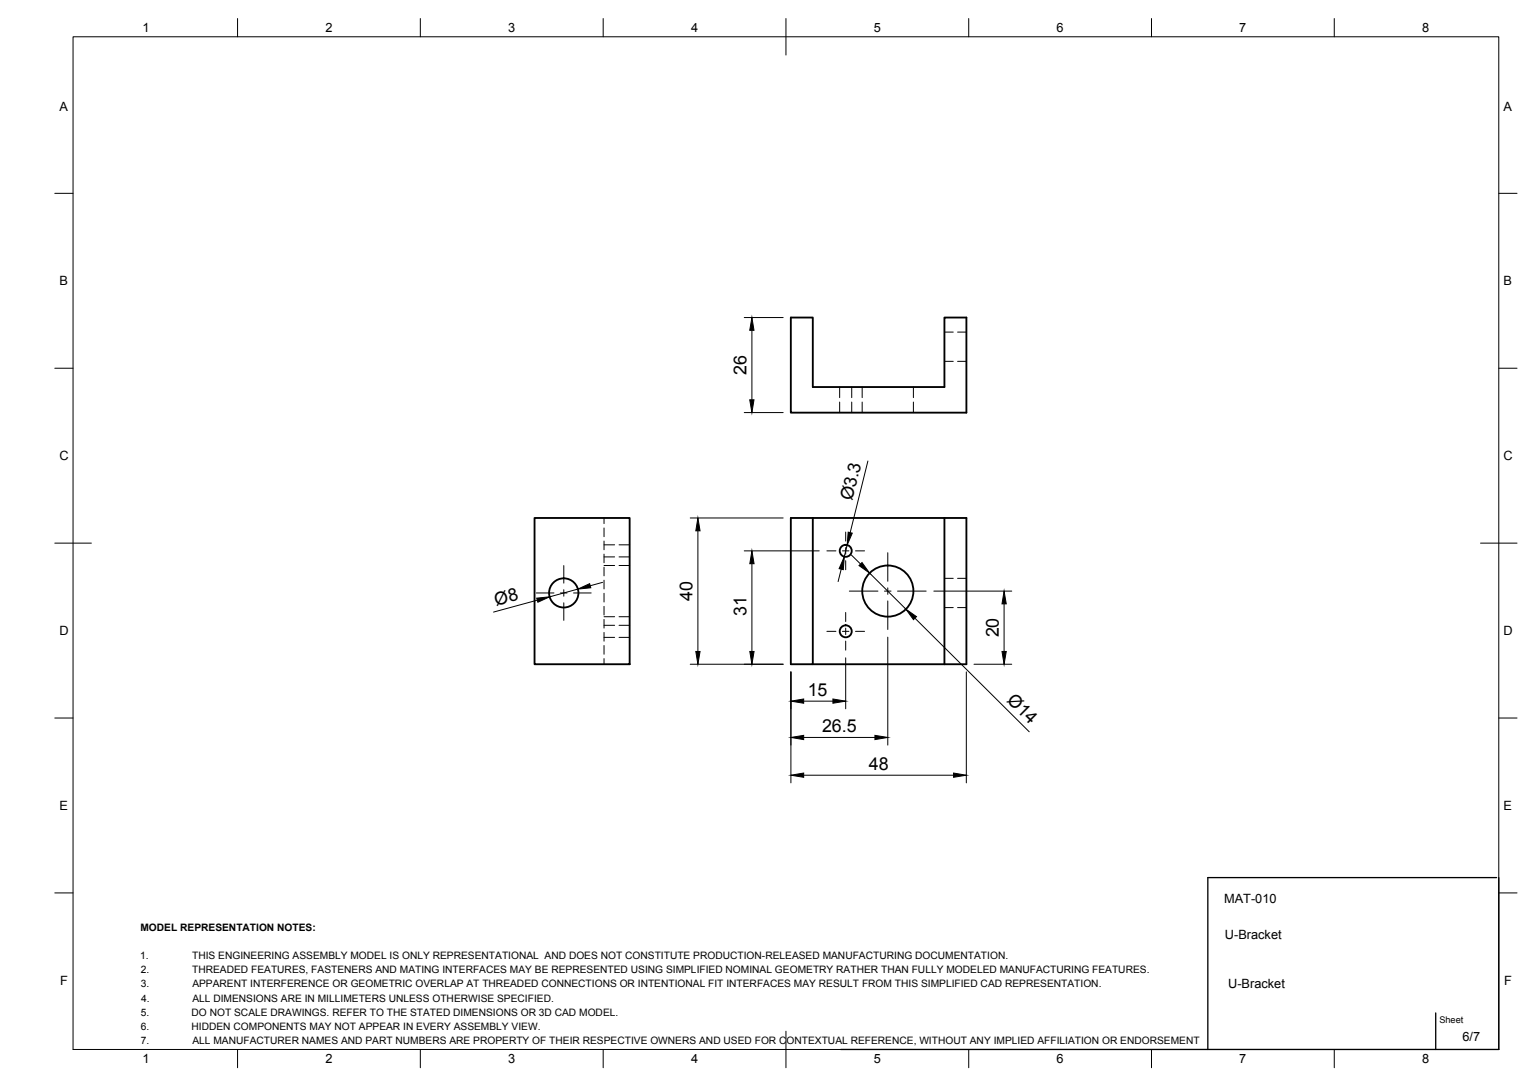
ISO-10303-21;
HEADER;
/* Generated by software containing ST-Developer
 * from STEP Tools, Inc. (www.steptools.com) 
 */

FILE_DESCRIPTION(
/* description */ ('STEP AP214'),
/* implementation_level */ '2;1');

FILE_NAME(
/* name */ 'U-Bracket.step',
/* time_stamp */ '2026-11-14T05:50:49-08:00',
/* author */ (''),
/* organization */ (''),
/* preprocessor_version */ 'ST-DEVELOPER v20.2',
/* originating_system */ 'Autodesk Translation Framework v15.17.0.0',
/* authorisation */ '');

FILE_SCHEMA (('AUTOMOTIVE_DESIGN { 1 0 10303 214 3 1 1 }'));
ENDSEC;

DATA;
#10=MECHANICAL_DESIGN_GEOMETRIC_PRESENTATION_REPRESENTATION('',(#161),#9903);
#147=SHAPE_REPRESENTATION_RELATIONSHIP('SRR','None',#9942,#154);
#154=ADVANCED_BREP_SHAPE_REPRESENTATION('',(#168),#9900);
#161=STYLED_ITEM('',(#9982),#168);
#168=MANIFOLD_SOLID_BREP('Body1',#2026);
#183=FACE_BOUND('',#426,.T.);
#184=FACE_BOUND('',#427,.T.);
#185=FACE_BOUND('',#428,.T.);
#186=FACE_BOUND('',#430,.T.);
#187=FACE_BOUND('',#435,.T.);
#188=FACE_BOUND('',#436,.T.);
#189=FACE_BOUND('',#437,.T.);
#190=FACE_BOUND('',#441,.T.);
#214=PLANE('',#2211);
#215=PLANE('',#2212);
#216=PLANE('',#2213);
#217=PLANE('',#2214);
#218=PLANE('',#2215);
#219=PLANE('',#2216);
#220=PLANE('',#2217);
#221=PLANE('',#2218);
#222=PLANE('',#2219);
#223=PLANE('',#2220);
#291=FACE_OUTER_BOUND('',#421,.T.);
#292=FACE_OUTER_BOUND('',#422,.T.);
#293=FACE_OUTER_BOUND('',#423,.T.);
#294=FACE_OUTER_BOUND('',#424,.T.);
#295=FACE_OUTER_BOUND('',#425,.T.);
#296=FACE_OUTER_BOUND('',#429,.T.);
#297=FACE_OUTER_BOUND('',#431,.T.);
#298=FACE_OUTER_BOUND('',#432,.T.);
#299=FACE_OUTER_BOUND('',#433,.T.);
#300=FACE_OUTER_BOUND('',#434,.T.);
#301=FACE_OUTER_BOUND('',#438,.T.);
#302=FACE_OUTER_BOUND('',#439,.T.);
#303=FACE_OUTER_BOUND('',#440,.T.);
#304=FACE_OUTER_BOUND('',#442,.T.);
#421=EDGE_LOOP('',(#1448,#1449,#1450,#1451));
#422=EDGE_LOOP('',(#1452,#1453,#1454,#1455));
#423=EDGE_LOOP('',(#1456,#1457,#1458,#1459));
#424=EDGE_LOOP('',(#1460,#1461,#1462,#1463));
#425=EDGE_LOOP('',(#1464,#1465,#1466,#1467));
#426=EDGE_LOOP('',(#1468));
#427=EDGE_LOOP('',(#1469));
#428=EDGE_LOOP('',(#1470));
#429=EDGE_LOOP('',(#1471,#1472,#1473,#1474));
#430=EDGE_LOOP('',(#1475));
#431=EDGE_LOOP('',(#1476,#1477,#1478,#1479,#1480,#1481,#1482,#1483));
#432=EDGE_LOOP('',(#1484,#1485,#1486,#1487));
#433=EDGE_LOOP('',(#1488,#1489,#1490,#1491,#1492,#1493,#1494,#1495));
#434=EDGE_LOOP('',(#1496,#1497,#1498,#1499));
#435=EDGE_LOOP('',(#1500));
#436=EDGE_LOOP('',(#1501));
#437=EDGE_LOOP('',(#1502));
#438=EDGE_LOOP('',(#1503,#1504,#1505,#1506));
#439=EDGE_LOOP('',(#1507,#1508,#1509,#1510));
#440=EDGE_LOOP('',(#1511,#1512,#1513,#1514));
#441=EDGE_LOOP('',(#1515));
#442=EDGE_LOOP('',(#1516,#1517,#1518,#1519));
#535=LINE('',#3038,#671);
#536=LINE('',#3044,#672);
#537=LINE('',#3050,#673);
#538=LINE('',#3056,#674);
#539=LINE('',#3061,#675);
#540=LINE('',#3063,#676);
#541=LINE('',#3065,#677);
#542=LINE('',#3066,#678);
#543=LINE('',#3070,#679);
#544=LINE('',#3072,#680);
#545=LINE('',#3074,#681);
#546=LINE('',#3075,#682);
#547=LINE('',#3078,#683);
#548=LINE('',#3080,#684);
#549=LINE('',#3082,#685);
#550=LINE('',#3083,#686);
#551=LINE('',#3085,#687);
#552=LINE('',#3086,#688);
#553=LINE('',#3089,#689);
#554=LINE('',#3091,#690);
#555=LINE('',#3092,#691);
#556=LINE('',#3094,#692);
#557=LINE('',#3096,#693);
#558=LINE('',#3097,#694);
#559=LINE('',#3099,#695);
#560=LINE('',#3100,#696);
#561=LINE('',#3103,#697);
#562=LINE('',#3106,#698);
#671=VECTOR('',#2528,4.);
#672=VECTOR('',#2535,1.64999999999999);
#673=VECTOR('',#2542,1.64999999999999);
#674=VECTOR('',#2549,7.);
#675=VECTOR('',#2554,1000.);
#676=VECTOR('',#2555,1000.);
#677=VECTOR('',#2556,1000.);
#678=VECTOR('',#2557,1000.);
#679=VECTOR('',#2560,1000.);
#680=VECTOR('',#2561,1000.);
#681=VECTOR('',#2562,1000.);
#682=VECTOR('',#2563,1000.);
#683=VECTOR('',#2566,1000.);
#684=VECTOR('',#2567,1000.);
#685=VECTOR('',#2568,1000.);
#686=VECTOR('',#2569,1000.);
#687=VECTOR('',#2570,1000.);
#688=VECTOR('',#2571,1000.);
#689=VECTOR('',#2574,1000.);
#690=VECTOR('',#2575,1000.);
#691=VECTOR('',#2576,1000.);
#692=VECTOR('',#2579,1000.);
#693=VECTOR('',#2580,1000.);
#694=VECTOR('',#2581,1000.);
#695=VECTOR('',#2582,1000.);
#696=VECTOR('',#2583,1000.);
#697=VECTOR('',#2588,1000.);
#698=VECTOR('',#2593,1000.);
#832=CIRCLE('',#2200,4.);
#833=CIRCLE('',#2201,4.);
#834=CIRCLE('',#2203,1.64999999999999);
#835=CIRCLE('',#2204,1.64999999999999);
#836=CIRCLE('',#2206,1.64999999999999);
#837=CIRCLE('',#2207,1.64999999999999);
#838=CIRCLE('',#2209,7.);
#839=CIRCLE('',#2210,7.);
#903=VERTEX_POINT('',#3035);
#904=VERTEX_POINT('',#3037);
#905=VERTEX_POINT('',#3041);
#906=VERTEX_POINT('',#3043);
#907=VERTEX_POINT('',#3047);
#908=VERTEX_POINT('',#3049);
#909=VERTEX_POINT('',#3053);
#910=VERTEX_POINT('',#3055);
#911=VERTEX_POINT('',#3059);
#912=VERTEX_POINT('',#3060);
#913=VERTEX_POINT('',#3062);
#914=VERTEX_POINT('',#3064);
#915=VERTEX_POINT('',#3068);
#916=VERTEX_POINT('',#3069);
#917=VERTEX_POINT('',#3071);
#918=VERTEX_POINT('',#3073);
#919=VERTEX_POINT('',#3077);
#920=VERTEX_POINT('',#3079);
#921=VERTEX_POINT('',#3081);
#922=VERTEX_POINT('',#3084);
#923=VERTEX_POINT('',#3088);
#924=VERTEX_POINT('',#3090);
#925=VERTEX_POINT('',#3095);
#926=VERTEX_POINT('',#3098);
#1105=EDGE_CURVE('',#903,#903,#832,.T.);
#1106=EDGE_CURVE('',#903,#904,#535,.T.);
#1107=EDGE_CURVE('',#904,#904,#833,.T.);
#1108=EDGE_CURVE('',#905,#905,#834,.T.);
#1109=EDGE_CURVE('',#905,#906,#536,.T.);
#1110=EDGE_CURVE('',#906,#906,#835,.T.);
#1111=EDGE_CURVE('',#907,#907,#836,.T.);
#1112=EDGE_CURVE('',#907,#908,#537,.T.);
#1113=EDGE_CURVE('',#908,#908,#837,.T.);
#1114=EDGE_CURVE('',#909,#909,#838,.T.);
#1115=EDGE_CURVE('',#909,#910,#538,.T.);
#1116=EDGE_CURVE('',#910,#910,#839,.T.);
#1117=EDGE_CURVE('',#911,#912,#539,.T.);
#1118=EDGE_CURVE('',#913,#912,#540,.T.);
#1119=EDGE_CURVE('',#913,#914,#541,.T.);
#1120=EDGE_CURVE('',#911,#914,#542,.T.);
#1121=EDGE_CURVE('',#915,#916,#543,.T.);
#1122=EDGE_CURVE('',#917,#916,#544,.T.);
#1123=EDGE_CURVE('',#918,#917,#545,.T.);
#1124=EDGE_CURVE('',#918,#915,#546,.T.);
#1125=EDGE_CURVE('',#916,#919,#547,.T.);
#1126=EDGE_CURVE('',#920,#919,#548,.T.);
#1127=EDGE_CURVE('',#921,#920,#549,.T.);
#1128=EDGE_CURVE('',#921,#914,#550,.T.);
#1129=EDGE_CURVE('',#922,#913,#551,.T.);
#1130=EDGE_CURVE('',#917,#922,#552,.T.);
#1131=EDGE_CURVE('',#919,#923,#553,.T.);
#1132=EDGE_CURVE('',#924,#923,#554,.T.);
#1133=EDGE_CURVE('',#920,#924,#555,.T.);
#1134=EDGE_CURVE('',#923,#915,#556,.T.);
#1135=EDGE_CURVE('',#925,#918,#557,.T.);
#1136=EDGE_CURVE('',#925,#912,#558,.T.);
#1137=EDGE_CURVE('',#926,#911,#559,.T.);
#1138=EDGE_CURVE('',#924,#926,#560,.T.);
#1139=EDGE_CURVE('',#926,#921,#561,.T.);
#1140=EDGE_CURVE('',#922,#925,#562,.T.);
#1448=ORIENTED_EDGE('',*,*,#1105,.F.);
#1449=ORIENTED_EDGE('',*,*,#1106,.T.);
#1450=ORIENTED_EDGE('',*,*,#1107,.T.);
#1451=ORIENTED_EDGE('',*,*,#1106,.F.);
#1452=ORIENTED_EDGE('',*,*,#1108,.T.);
#1453=ORIENTED_EDGE('',*,*,#1109,.T.);
#1454=ORIENTED_EDGE('',*,*,#1110,.T.);
#1455=ORIENTED_EDGE('',*,*,#1109,.F.);
#1456=ORIENTED_EDGE('',*,*,#1111,.T.);
#1457=ORIENTED_EDGE('',*,*,#1112,.T.);
#1458=ORIENTED_EDGE('',*,*,#1113,.T.);
#1459=ORIENTED_EDGE('',*,*,#1112,.F.);
#1460=ORIENTED_EDGE('',*,*,#1114,.T.);
#1461=ORIENTED_EDGE('',*,*,#1115,.T.);
#1462=ORIENTED_EDGE('',*,*,#1116,.T.);
#1463=ORIENTED_EDGE('',*,*,#1115,.F.);
#1464=ORIENTED_EDGE('',*,*,#1117,.T.);
#1465=ORIENTED_EDGE('',*,*,#1118,.F.);
#1466=ORIENTED_EDGE('',*,*,#1119,.T.);
#1467=ORIENTED_EDGE('',*,*,#1120,.F.);
#1468=ORIENTED_EDGE('',*,*,#1108,.F.);
#1469=ORIENTED_EDGE('',*,*,#1111,.F.);
#1470=ORIENTED_EDGE('',*,*,#1114,.F.);
#1471=ORIENTED_EDGE('',*,*,#1121,.T.);
#1472=ORIENTED_EDGE('',*,*,#1122,.F.);
#1473=ORIENTED_EDGE('',*,*,#1123,.F.);
#1474=ORIENTED_EDGE('',*,*,#1124,.T.);
#1475=ORIENTED_EDGE('',*,*,#1107,.F.);
#1476=ORIENTED_EDGE('',*,*,#1125,.T.);
#1477=ORIENTED_EDGE('',*,*,#1126,.F.);
#1478=ORIENTED_EDGE('',*,*,#1127,.F.);
#1479=ORIENTED_EDGE('',*,*,#1128,.T.);
#1480=ORIENTED_EDGE('',*,*,#1119,.F.);
#1481=ORIENTED_EDGE('',*,*,#1129,.F.);
#1482=ORIENTED_EDGE('',*,*,#1130,.F.);
#1483=ORIENTED_EDGE('',*,*,#1122,.T.);
#1484=ORIENTED_EDGE('',*,*,#1131,.T.);
#1485=ORIENTED_EDGE('',*,*,#1132,.F.);
#1486=ORIENTED_EDGE('',*,*,#1133,.F.);
#1487=ORIENTED_EDGE('',*,*,#1126,.T.);
#1488=ORIENTED_EDGE('',*,*,#1134,.T.);
#1489=ORIENTED_EDGE('',*,*,#1124,.F.);
#1490=ORIENTED_EDGE('',*,*,#1135,.F.);
#1491=ORIENTED_EDGE('',*,*,#1136,.T.);
#1492=ORIENTED_EDGE('',*,*,#1117,.F.);
#1493=ORIENTED_EDGE('',*,*,#1137,.F.);
#1494=ORIENTED_EDGE('',*,*,#1138,.F.);
#1495=ORIENTED_EDGE('',*,*,#1132,.T.);
#1496=ORIENTED_EDGE('',*,*,#1121,.F.);
#1497=ORIENTED_EDGE('',*,*,#1134,.F.);
#1498=ORIENTED_EDGE('',*,*,#1131,.F.);
#1499=ORIENTED_EDGE('',*,*,#1125,.F.);
#1500=ORIENTED_EDGE('',*,*,#1110,.F.);
#1501=ORIENTED_EDGE('',*,*,#1113,.F.);
#1502=ORIENTED_EDGE('',*,*,#1116,.F.);
#1503=ORIENTED_EDGE('',*,*,#1120,.T.);
#1504=ORIENTED_EDGE('',*,*,#1128,.F.);
#1505=ORIENTED_EDGE('',*,*,#1139,.F.);
#1506=ORIENTED_EDGE('',*,*,#1137,.T.);
#1507=ORIENTED_EDGE('',*,*,#1133,.T.);
#1508=ORIENTED_EDGE('',*,*,#1138,.T.);
#1509=ORIENTED_EDGE('',*,*,#1139,.T.);
#1510=ORIENTED_EDGE('',*,*,#1127,.T.);
#1511=ORIENTED_EDGE('',*,*,#1118,.T.);
#1512=ORIENTED_EDGE('',*,*,#1136,.F.);
#1513=ORIENTED_EDGE('',*,*,#1140,.F.);
#1514=ORIENTED_EDGE('',*,*,#1129,.T.);
#1515=ORIENTED_EDGE('',*,*,#1105,.T.);
#1516=ORIENTED_EDGE('',*,*,#1123,.T.);
#1517=ORIENTED_EDGE('',*,*,#1130,.T.);
#1518=ORIENTED_EDGE('',*,*,#1140,.T.);
#1519=ORIENTED_EDGE('',*,*,#1135,.T.);
#1870=CYLINDRICAL_SURFACE('',#2199,4.);
#1871=CYLINDRICAL_SURFACE('',#2202,1.64999999999999);
#1872=CYLINDRICAL_SURFACE('',#2205,1.64999999999999);
#1873=CYLINDRICAL_SURFACE('',#2208,7.);
#1943=ADVANCED_FACE('',(#291),#1870,.F.);
#1944=ADVANCED_FACE('',(#292),#1871,.F.);
#1945=ADVANCED_FACE('',(#293),#1872,.F.);
#1946=ADVANCED_FACE('',(#294),#1873,.F.);
#1947=ADVANCED_FACE('',(#295,#183,#184,#185),#214,.T.);
#1948=ADVANCED_FACE('',(#296,#186),#215,.F.);
#1949=ADVANCED_FACE('',(#297),#216,.F.);
#1950=ADVANCED_FACE('',(#298),#217,.F.);
#1951=ADVANCED_FACE('',(#299),#218,.F.);
#1952=ADVANCED_FACE('',(#300,#187,#188,#189),#219,.F.);
#1953=ADVANCED_FACE('',(#301),#220,.F.);
#1954=ADVANCED_FACE('',(#302),#221,.T.);
#1955=ADVANCED_FACE('',(#303,#190),#222,.F.);
#1956=ADVANCED_FACE('',(#304),#223,.F.);
#2026=CLOSED_SHELL('',(#1943,#1944,#1945,#1946,#1947,#1948,#1949,#1950,
#1951,#1952,#1953,#1954,#1955,#1956));
#2198=AXIS2_PLACEMENT_3D('',#3033,#2522,#2523);
#2199=AXIS2_PLACEMENT_3D('',#3034,#2524,#2525);
#2200=AXIS2_PLACEMENT_3D('',#3036,#2526,#2527);
#2201=AXIS2_PLACEMENT_3D('',#3039,#2529,#2530);
#2202=AXIS2_PLACEMENT_3D('',#3040,#2531,#2532);
#2203=AXIS2_PLACEMENT_3D('',#3042,#2533,#2534);
#2204=AXIS2_PLACEMENT_3D('',#3045,#2536,#2537);
#2205=AXIS2_PLACEMENT_3D('',#3046,#2538,#2539);
#2206=AXIS2_PLACEMENT_3D('',#3048,#2540,#2541);
#2207=AXIS2_PLACEMENT_3D('',#3051,#2543,#2544);
#2208=AXIS2_PLACEMENT_3D('',#3052,#2545,#2546);
#2209=AXIS2_PLACEMENT_3D('',#3054,#2547,#2548);
#2210=AXIS2_PLACEMENT_3D('',#3057,#2550,#2551);
#2211=AXIS2_PLACEMENT_3D('',#3058,#2552,#2553);
#2212=AXIS2_PLACEMENT_3D('',#3067,#2558,#2559);
#2213=AXIS2_PLACEMENT_3D('',#3076,#2564,#2565);
#2214=AXIS2_PLACEMENT_3D('',#3087,#2572,#2573);
#2215=AXIS2_PLACEMENT_3D('',#3093,#2577,#2578);
#2216=AXIS2_PLACEMENT_3D('',#3101,#2584,#2585);
#2217=AXIS2_PLACEMENT_3D('',#3102,#2586,#2587);
#2218=AXIS2_PLACEMENT_3D('',#3104,#2589,#2590);
#2219=AXIS2_PLACEMENT_3D('',#3105,#2591,#2592);
#2220=AXIS2_PLACEMENT_3D('',#3107,#2594,#2595);
#2522=DIRECTION('axis',(0.,0.,1.));
#2523=DIRECTION('refdir',(1.,0.,0.));
#2524=DIRECTION('center_axis',(0.,-1.,0.));
#2525=DIRECTION('ref_axis',(0.,0.,-1.));
#2526=DIRECTION('center_axis',(0.,-1.,0.));
#2527=DIRECTION('ref_axis',(0.,0.,-1.));
#2528=DIRECTION('',(0.,-1.,0.));
#2529=DIRECTION('center_axis',(0.,-1.,0.));
#2530=DIRECTION('ref_axis',(0.,0.,-1.));
#2531=DIRECTION('center_axis',(0.,0.,-1.));
#2532=DIRECTION('ref_axis',(-1.,0.,0.));
#2533=DIRECTION('center_axis',(0.,0.,1.));
#2534=DIRECTION('ref_axis',(1.,0.,0.));
#2535=DIRECTION('',(0.,0.,-1.));
#2536=DIRECTION('center_axis',(0.,0.,-1.));
#2537=DIRECTION('ref_axis',(-1.,0.,0.));
#2538=DIRECTION('center_axis',(0.,0.,-1.));
#2539=DIRECTION('ref_axis',(-1.,0.,0.));
#2540=DIRECTION('center_axis',(0.,0.,1.));
#2541=DIRECTION('ref_axis',(1.,0.,0.));
#2542=DIRECTION('',(0.,0.,-1.));
#2543=DIRECTION('center_axis',(0.,0.,-1.));
#2544=DIRECTION('ref_axis',(-1.,0.,0.));
#2545=DIRECTION('center_axis',(0.,0.,-1.));
#2546=DIRECTION('ref_axis',(-1.,0.,0.));
#2547=DIRECTION('center_axis',(0.,0.,1.));
#2548=DIRECTION('ref_axis',(1.,0.,0.));
#2549=DIRECTION('',(0.,0.,-1.));
#2550=DIRECTION('center_axis',(0.,0.,-1.));
#2551=DIRECTION('ref_axis',(-1.,0.,0.));
#2552=DIRECTION('center_axis',(0.,0.,1.));
#2553=DIRECTION('ref_axis',(1.,0.,0.));
#2554=DIRECTION('',(0.,-1.,0.));
#2555=DIRECTION('',(-1.,0.,0.));
#2556=DIRECTION('',(0.,1.,0.));
#2557=DIRECTION('',(1.,0.,0.));
#2558=DIRECTION('center_axis',(0.,1.,0.));
#2559=DIRECTION('ref_axis',(0.,0.,1.));
#2560=DIRECTION('',(1.,0.,0.));
#2561=DIRECTION('',(0.,0.,-1.));
#2562=DIRECTION('',(1.,0.,0.));
#2563=DIRECTION('',(0.,0.,-1.));
#2564=DIRECTION('center_axis',(-1.,0.,0.));
#2565=DIRECTION('ref_axis',(0.,0.,1.));
#2566=DIRECTION('',(0.,1.,0.));
#2567=DIRECTION('',(0.,0.,-1.));
#2568=DIRECTION('',(0.,1.,0.));
#2569=DIRECTION('',(0.,0.,-1.));
#2570=DIRECTION('',(0.,0.,-1.));
#2571=DIRECTION('',(0.,1.,0.));
#2572=DIRECTION('center_axis',(8.67361737988404E-17,-1.,0.));
#2573=DIRECTION('ref_axis',(1.,8.67361737988404E-17,0.));
#2574=DIRECTION('',(-1.,-8.67361737988404E-17,0.));
#2575=DIRECTION('',(0.,0.,-1.));
#2576=DIRECTION('',(-1.,-8.67361737988404E-17,0.));
#2577=DIRECTION('center_axis',(1.,0.,0.));
#2578=DIRECTION('ref_axis',(0.,0.,-1.));
#2579=DIRECTION('',(0.,-1.,0.));
#2580=DIRECTION('',(0.,-1.,0.));
#2581=DIRECTION('',(0.,0.,-1.));
#2582=DIRECTION('',(0.,0.,-1.));
#2583=DIRECTION('',(0.,-1.,0.));
#2584=DIRECTION('center_axis',(0.,0.,1.));
#2585=DIRECTION('ref_axis',(1.,0.,0.));
#2586=DIRECTION('center_axis',(0.,1.,0.));
#2587=DIRECTION('ref_axis',(0.,0.,1.));
#2588=DIRECTION('',(1.,0.,0.));
#2589=DIRECTION('center_axis',(0.,0.,1.));
#2590=DIRECTION('ref_axis',(1.,0.,0.));
#2591=DIRECTION('center_axis',(0.,-1.,0.));
#2592=DIRECTION('ref_axis',(0.,0.,-1.));
#2593=DIRECTION('',(-1.,0.,0.));
#2594=DIRECTION('center_axis',(0.,0.,-1.));
#2595=DIRECTION('ref_axis',(-1.,0.,0.));
#3033=CARTESIAN_POINT('',(0.,0.,0.));
#3034=CARTESIAN_POINT('Origin',(-0.506247771123191,-14.,18.0160339934195));
#3035=CARTESIAN_POINT('',(-0.506247771123192,-18.,22.0160339934195));
#3036=CARTESIAN_POINT('Origin',(-0.506247771123191,-18.,18.0160339934195));
#3037=CARTESIAN_POINT('',(-0.506247771123192,-24.,22.0160339934195));
#3038=CARTESIAN_POINT('',(-0.506247771123192,-14.,22.0160339934195));
#3039=CARTESIAN_POINT('Origin',(-0.506247771123191,-24.,18.0160339934195));
#3040=CARTESIAN_POINT('Origin',(-11.,9.00000000000001,0.));
#3041=CARTESIAN_POINT('',(-9.35000000000001,9.00000000000001,7.));
#3042=CARTESIAN_POINT('Origin',(-11.,9.00000000000001,7.));
#3043=CARTESIAN_POINT('',(-9.35000000000001,9.00000000000001,-1.35323471305782E-15));
#3044=CARTESIAN_POINT('',(-9.35000000000001,9.00000000000001,0.));
#3045=CARTESIAN_POINT('Origin',(-11.,9.00000000000001,-1.35323471305782E-15));
#3046=CARTESIAN_POINT('Origin',(11.,9.,0.));
#3047=CARTESIAN_POINT('',(12.65,9.,7.));
#3048=CARTESIAN_POINT('Origin',(11.,9.,7.));
#3049=CARTESIAN_POINT('',(12.65,9.,-1.35323471305782E-15));
#3050=CARTESIAN_POINT('',(12.65,9.,0.));
#3051=CARTESIAN_POINT('Origin',(11.,9.,-1.35323471305782E-15));
#3052=CARTESIAN_POINT('Origin',(0.,-2.5,9.99999999999999));
#3053=CARTESIAN_POINT('',(7.,-2.5,7.));
#3054=CARTESIAN_POINT('Origin',(0.,-2.5,7.));
#3055=CARTESIAN_POINT('',(7.,-2.5,-1.11022302462516E-15));
#3056=CARTESIAN_POINT('',(7.,-2.5,9.99999999999999));
#3057=CARTESIAN_POINT('Origin',(0.,-2.5,0.));
#3058=CARTESIAN_POINT('Origin',(0.,0.,7.));
#3059=CARTESIAN_POINT('',(-20.,18.,7.));
#3060=CARTESIAN_POINT('',(-20.,-18.,7.));
#3061=CARTESIAN_POINT('',(-20.,24.,7.));
#3062=CARTESIAN_POINT('',(20.,-18.,7.));
#3063=CARTESIAN_POINT('',(-20.,-18.,7.));
#3064=CARTESIAN_POINT('',(20.,18.,7.));
#3065=CARTESIAN_POINT('',(20.,-24.,7.));
#3066=CARTESIAN_POINT('',(-20.,18.,7.));
#3067=CARTESIAN_POINT('Origin',(2.93915231795365E-15,-24.,7.));
#3068=CARTESIAN_POINT('',(-20.,-24.,0.));
#3069=CARTESIAN_POINT('',(20.,-24.,0.));
#3070=CARTESIAN_POINT('',(2.93915231795365E-15,-24.,0.));
#3071=CARTESIAN_POINT('',(20.,-24.,26.));
#3072=CARTESIAN_POINT('',(20.,-24.,7.));
#3073=CARTESIAN_POINT('',(-20.,-24.,26.));
#3074=CARTESIAN_POINT('',(20.,-24.,26.));
#3075=CARTESIAN_POINT('',(-20.,-24.,7.));
#3076=CARTESIAN_POINT('Origin',(20.,-24.,7.));
#3077=CARTESIAN_POINT('',(20.,24.,0.));
#3078=CARTESIAN_POINT('',(20.,-24.,0.));
#3079=CARTESIAN_POINT('',(20.,24.,26.));
#3080=CARTESIAN_POINT('',(20.,24.,7.));
#3081=CARTESIAN_POINT('',(20.,18.,26.));
#3082=CARTESIAN_POINT('',(20.,18.,26.));
#3083=CARTESIAN_POINT('',(20.,18.,26.));
#3084=CARTESIAN_POINT('',(20.,-18.,26.));
#3085=CARTESIAN_POINT('',(20.,-18.,26.));
#3086=CARTESIAN_POINT('',(20.,-18.,26.));
#3087=CARTESIAN_POINT('Origin',(20.,24.,7.));
#3088=CARTESIAN_POINT('',(-20.,24.,0.));
#3089=CARTESIAN_POINT('',(20.,24.,0.));
#3090=CARTESIAN_POINT('',(-20.,24.,26.));
#3091=CARTESIAN_POINT('',(-20.,24.,7.));
#3092=CARTESIAN_POINT('',(20.,24.,26.));
#3093=CARTESIAN_POINT('Origin',(-20.,24.,7.));
#3094=CARTESIAN_POINT('',(-20.,24.,0.));
#3095=CARTESIAN_POINT('',(-20.,-18.,26.));
#3096=CARTESIAN_POINT('',(-20.,-24.,26.));
#3097=CARTESIAN_POINT('',(-20.,-18.,26.));
#3098=CARTESIAN_POINT('',(-20.,18.,26.));
#3099=CARTESIAN_POINT('',(-20.,18.,26.));
#3100=CARTESIAN_POINT('',(-20.,24.,26.));
#3101=CARTESIAN_POINT('Origin',(0.,0.,0.));
#3102=CARTESIAN_POINT('Origin',(-20.,18.,26.));
#3103=CARTESIAN_POINT('',(-20.,18.,26.));
#3104=CARTESIAN_POINT('Origin',(0.,0.,26.));
#3105=CARTESIAN_POINT('Origin',(-20.,-18.,26.));
#3106=CARTESIAN_POINT('',(-20.,-18.,26.));
#3107=CARTESIAN_POINT('Origin',(0.,0.,26.));
#9891=UNCERTAINTY_MEASURE_WITH_UNIT(LENGTH_MEASURE(0.01),#9904,
'DISTANCE_ACCURACY_VALUE',
'Maximum model space distance between geometric entities at asserted c
onnectivities');
#9894=UNCERTAINTY_MEASURE_WITH_UNIT(LENGTH_MEASURE(0.01),#9904,
'DISTANCE_ACCURACY_VALUE',
'Maximum model space distance between geometric entities at asserted c
onnectivities');
#9900=(
GEOMETRIC_REPRESENTATION_CONTEXT(3)
GLOBAL_UNCERTAINTY_ASSIGNED_CONTEXT((#9891))
GLOBAL_UNIT_ASSIGNED_CONTEXT((#9904,#9906,#9907))
REPRESENTATION_CONTEXT('','3D')
);
#9903=(
GEOMETRIC_REPRESENTATION_CONTEXT(3)
GLOBAL_UNCERTAINTY_ASSIGNED_CONTEXT((#9894))
GLOBAL_UNIT_ASSIGNED_CONTEXT((#9904,#9906,#9907))
REPRESENTATION_CONTEXT('','3D')
);
#9904=(
LENGTH_UNIT()
NAMED_UNIT(*)
SI_UNIT(.MILLI.,.METRE.)
);
#9906=(
NAMED_UNIT(*)
PLANE_ANGLE_UNIT()
SI_UNIT($,.RADIAN.)
);
#9907=(
NAMED_UNIT(*)
SI_UNIT($,.STERADIAN.)
SOLID_ANGLE_UNIT()
);
#9913=SHAPE_DEFINITION_REPRESENTATION(#9921,#9942);
#9921=PRODUCT_DEFINITION_SHAPE('',$,#9951);
#9942=SHAPE_REPRESENTATION('',(#2198),#9900);
#9945=PRODUCT_DEFINITION_CONTEXT('part definition',#9971,'design');
#9951=PRODUCT_DEFINITION('U-Bracket','U-Bracket',#9959,#9945);
#9959=PRODUCT_DEFINITION_FORMATION('',$,#9978);
#9971=APPLICATION_CONTEXT(
'Core Data for Automotive Mechanical Design Process');
#9972=PRODUCT_CONTEXT('part definition',#9971,'mechanical');
#9978=PRODUCT('U-Bracket','U-Bracket',$,(#9972));
#9982=PRESENTATION_STYLE_ASSIGNMENT((#9987));
#9987=SURFACE_STYLE_USAGE(.BOTH.,#9992);
#9992=SURFACE_SIDE_STYLE('',(#9997));
#9997=SURFACE_STYLE_FILL_AREA(#10002);
#10002=FILL_AREA_STYLE('Opaque(97,158,199)',(#10007));
#10007=FILL_AREA_STYLE_COLOUR('Opaque(97,158,199)',#10012);
#10012=COLOUR_RGB('Opaque(97,158,199)',0.380392156862745,0.619607843137255,
0.780392156862745);
ENDSEC;
END-ISO-10303-21;
